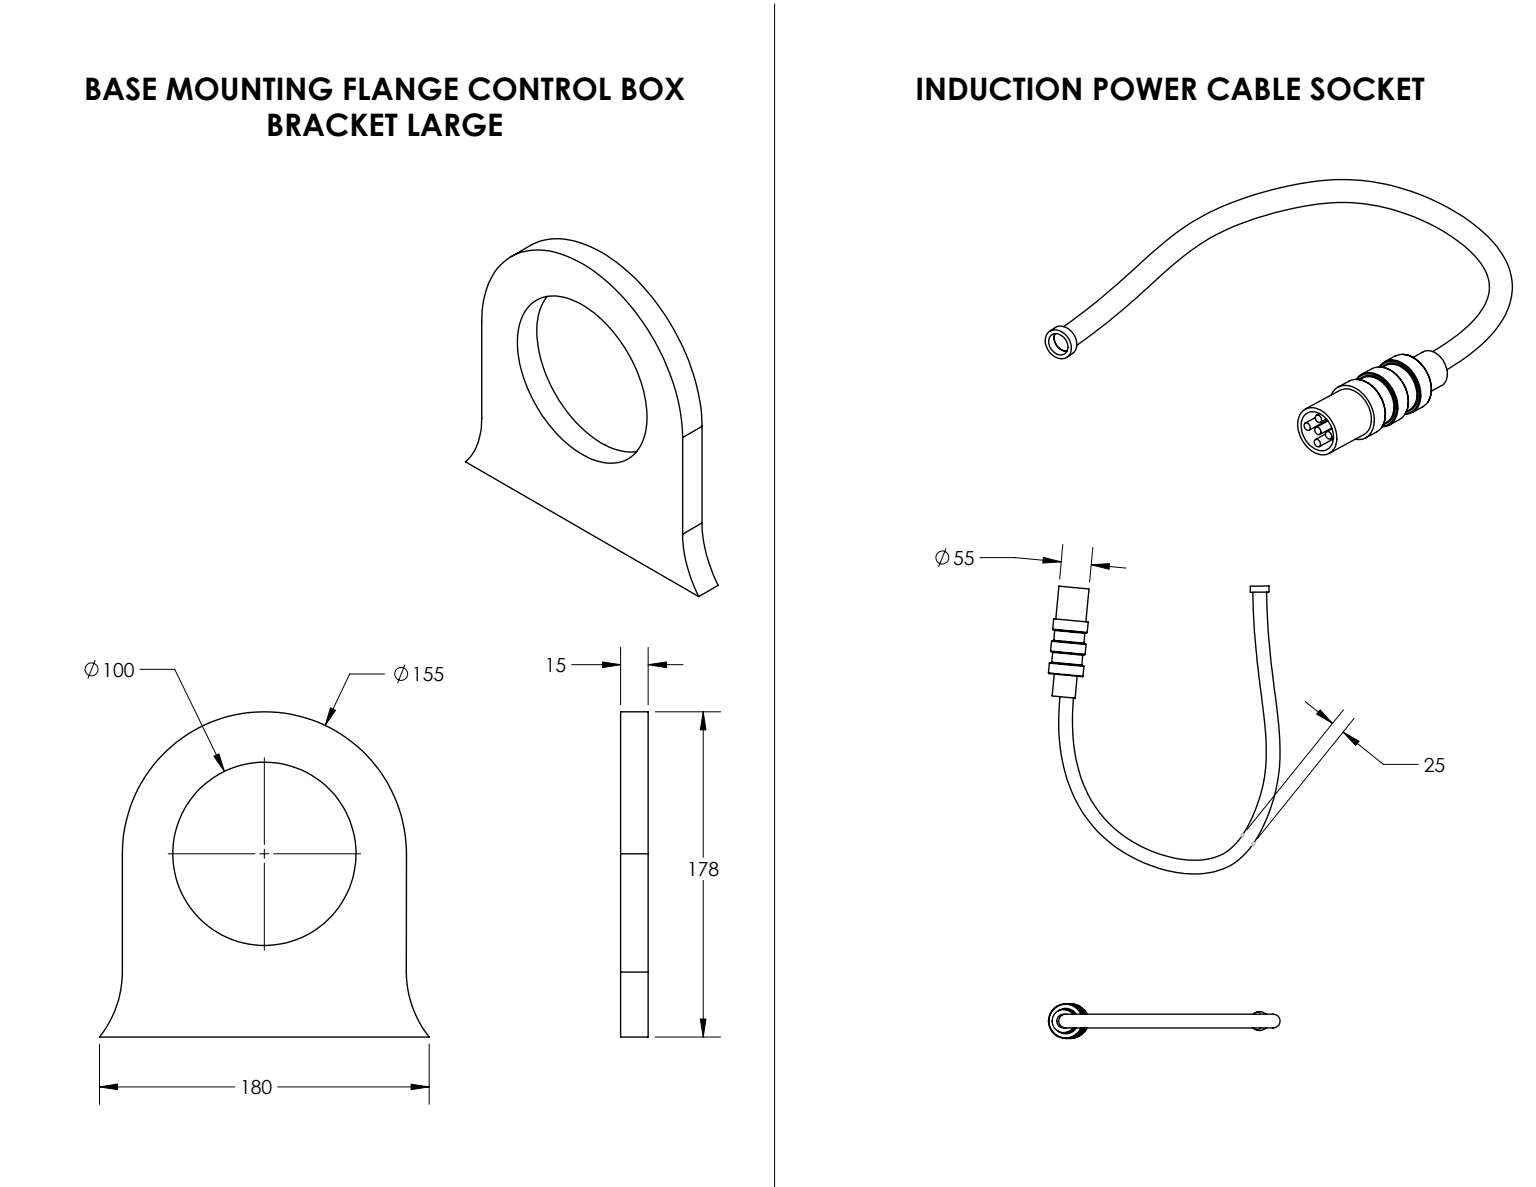
ISO-10303-21;
HEADER;
FILE_DESCRIPTION (('STEP AP214'),
    '1' );
FILE_NAME ('Base Mounting Flange Control Box Bracket large.step',
    '2026-10-28T18:30:06',
    ( '' ),
    ( '' ),
    'SwSTEP 2.0',
    'SolidWorks 2024',
    '' );
FILE_SCHEMA (( 'AUTOMOTIVE_DESIGN' ));
ENDSEC;

DATA;
#28=VECTOR ( 'NONE', #1957, 1000.000000000000114 ) ;
#31=DIRECTION ( 'NONE',  ( 0.000000000000000000, 1.000000000000000000, 0.000000000000000000 ) ) ;
#39=ORIENTED_EDGE ( 'NONE', *, *, #4059, .T. ) ;
#42=AXIS2_PLACEMENT_3D ( 'NONE', #2101, #4638, #4224 ) ;
#54=SHAPE_REPRESENTATION_RELATIONSHIP ( 'NONE' , 'NONE' ,  #825, #4179 ) ;
#57=EDGE_CURVE ( 'NONE', #2668, #1622, #1040, .T. ) ;
#90=ADVANCED_FACE ( 'NONE', ( #1835, #4370 ), #3525, .T. ) ;
#123=CARTESIAN_POINT ( 'NONE',  ( 29.23877717791899400, 15.00000000000001421, -10.40386589866737488 ) ) ;
#142=FACE_OUTER_BOUND ( 'NONE', #4109, .T. ) ;
#153=VECTOR ( 'NONE', #3723, 1000.000000000000000 ) ;
#184=DIRECTION ( 'NONE',  ( 0.000000000000000000, -1.000000000000000000, 0.000000000000000000 ) ) ;
#185=DIRECTION ( 'NONE',  ( -5.551115123125785167E-17, 0.000000000000000000, -1.000000000000000000 ) ) ;
#197=VECTOR ( 'NONE', #4836, 1000.000000000000000 ) ;
#202=DIRECTION ( 'NONE',  ( 6.938893903907233308E-17, 0.000000000000000000, 1.000000000000000000 ) ) ;
#208=CARTESIAN_POINT ( 'NONE',  ( 102.9433289385998478, 15.00000000000001421, 135.9081080810072137 ) ) ;
#225=DIRECTION ( 'NONE',  ( 6.938893903907233308E-17, 0.000000000000000000, 1.000000000000000000 ) ) ;
#226=EDGE_CURVE ( 'NONE', #1002, #2668, #2706, .T. ) ;
#228=EDGE_CURVE ( 'NONE', #5171, #2162, #3633, .T. ) ;
#243=CARTESIAN_POINT ( 'NONE',  ( -66.30461487616335603, 15.00000000000001421, 161.8139267001887447 ) ) ;
#269=DIRECTION ( 'NONE',  ( 0.000000000000000000, 0.000000000000000000, -1.000000000000000000 ) ) ;
#285=AXIS2_PLACEMENT_3D ( 'NONE', #400, #2072, #1734 ) ;
#298=EDGE_CURVE ( 'NONE', #1751, #1002, #1747, .T. ) ;
#323=ORIENTED_EDGE ( 'NONE', *, *, #228, .T. ) ;
#334=EDGE_CURVE ( 'NONE', #2890, #2427, #2526, .T. ) ;
#367=DIRECTION ( 'NONE',  ( 0.000000000000000000, 0.000000000000000000, -1.000000000000000000 ) ) ;
#368=DIRECTION ( 'NONE',  ( 0.000000000000000000, -1.000000000000000000, 0.000000000000000000 ) ) ;
#400=CARTESIAN_POINT ( 'NONE',  ( 29.23877717791899755, 15.00000000000001421, 67.09613410133263756 ) ) ;
#407=DIRECTION ( 'NONE',  ( 0.000000000000000000, 1.000000000000000000, 0.000000000000000000 ) ) ;
#419=CARTESIAN_POINT ( 'NONE',  ( 29.23877717791899755, 15.00000000000001421, 67.09613410133263756 ) ) ;
#456=CARTESIAN_POINT ( 'NONE',  ( 29.23877717791900466, 15.00000000000001421, 117.0961341013325949 ) ) ;
#458=FACE_OUTER_BOUND ( 'NONE', #2128, .T. ) ;
#460=EDGE_CURVE ( 'NONE', #2116, #2668, #3869, .T. ) ;
#474=ORIENTED_EDGE ( 'NONE', *, *, #2339, .F. ) ;
#500=ORIENTED_EDGE ( 'NONE', *, *, #5068, .F. ) ;
#519=ORIENTED_EDGE ( 'NONE', *, *, #1198, .T. ) ;
#529=CARTESIAN_POINT ( 'NONE',  ( 29.23877717791899755, 15.00000000000001421, 67.09613410133263756 ) ) ;
#530=EDGE_CURVE ( 'NONE', #606, #5098, #1451, .T. ) ;
#582=CYLINDRICAL_SURFACE ( 'NONE', #4512, 77.49999999999998579 ) ;
#590=ORIENTED_EDGE ( 'NONE', *, *, #226, .F. ) ;
#597=DIRECTION ( 'NONE',  ( 0.05689159511111528678, 0.000000000000000000, -0.9983803615885644689 ) ) ;
#602=ORIENTED_EDGE ( 'NONE', *, *, #2737, .T. ) ;
#604=DIRECTION ( 'NONE',  ( -4.476705744456277327E-17, 0.000000000000000000, -1.000000000000000000 ) ) ;
#606=VERTEX_POINT ( 'NONE', #3188 ) ;
#608=CARTESIAN_POINT ( 'NONE',  ( 29.23877717791899755, 15.00000000000001421, 67.09613410133263756 ) ) ;
#625=ORIENTED_EDGE ( 'NONE', *, *, #460, .F. ) ;
#643=ORIENTED_EDGE ( 'NONE', *, *, #2742, .F. ) ;
#663=DIRECTION ( 'NONE',  ( 0.000000000000000000, -1.000000000000000000, -0.000000000000000000 ) ) ;
#706=EDGE_LOOP ( 'NONE', ( #2402, #1700, #643, #922 ) ) ;
#708=EDGE_LOOP ( 'NONE', ( #3884, #2629, #2702, #889 ) ) ;
#715=CIRCLE ( 'NONE', #1161, 56.63911695420845405 ) ;
#746=FACE_BOUND ( 'NONE', #3021, .T. ) ;
#775=UNCERTAINTY_MEASURE_WITH_UNIT (LENGTH_MEASURE( 1.000000000000000082E-05 ), #2148, 'distance_accuracy_value', 'NONE');
#796=EDGE_CURVE ( 'NONE', #2890, #3556, #4181, .T. ) ;
#802=DIRECTION ( 'NONE',  ( -6.938893903907233308E-17, 0.000000000000000000, -1.000000000000000000 ) ) ;
#810=DIRECTION ( 'NONE',  ( 0.000000000000000000, -1.000000000000000000, 0.000000000000000000 ) ) ;
#825=SHAPE_REPRESENTATION ( 'Base Mounting Flange Control Box Bracket large', ( #2926 ), #1963 ) ;
#835=PRODUCT ( 'Base Mounting Flange Control Box Bracket large', 'Base Mounting Flange Control Box Bracket large', '', ( #4423 ) ) ;
#845=DIRECTION ( 'NONE',  ( 4.476705744456277327E-17, 0.000000000000000000, 1.000000000000000000 ) ) ;
#889=ORIENTED_EDGE ( 'NONE', *, *, #4257, .F. ) ;
#890=ORIENTED_EDGE ( 'NONE', *, *, #5426, .F. ) ;
#905=AXIS2_PLACEMENT_3D ( 'NONE', #4213, #4650, #2237 ) ;
#914=AXIS2_PLACEMENT_3D ( 'NONE', #2171, #3387, #4641 ) ;
#922=ORIENTED_EDGE ( 'NONE', *, *, #4994, .F. ) ;
#935=ADVANCED_FACE ( 'NONE', ( #3434 ), #5172, .F. ) ;
#937=CARTESIAN_POINT ( 'NONE',  ( 29.23877717791899400, 0.000000000000000000, -10.40386589866737488 ) ) ;
#948=DIRECTION ( 'NONE',  ( 0.05689159511111530065, 0.000000000000000000, -0.9983803615885645799 ) ) ;
#959=DIRECTION ( 'NONE',  ( 0.000000000000000000, 0.000000000000000000, 1.000000000000000000 ) ) ;
#1002=VERTEX_POINT ( 'NONE', #1518 ) ;
#1006=VECTOR ( 'NONE', #5359, 1000.000000000000000 ) ;
#1009=AXIS2_PLACEMENT_3D ( 'NONE', #4115, #368, #802 ) ;
#1016=DIRECTION ( 'NONE',  ( 0.000000000000000000, -1.000000000000000000, -0.000000000000000000 ) ) ;
#1040=LINE ( 'NONE', #1062, #2701 ) ;
#1044=ORIENTED_EDGE ( 'NONE', *, *, #796, .F. ) ;
#1055=AXIS2_PLACEMENT_3D ( 'NONE', #1273, #3419, #2996 ) ;
#1062=CARTESIAN_POINT ( 'NONE',  ( 102.9433289385998478, 0.000000000000000000, 135.9081080810072137 ) ) ;
#1084=DIRECTION ( 'NONE',  ( 0.000000000000000000, -1.000000000000000000, 0.000000000000000000 ) ) ;
#1103=DIRECTION ( 'NONE',  ( 0.000000000000000000, 1.000000000000000000, 0.000000000000000000 ) ) ;
#1137=CARTESIAN_POINT ( 'NONE',  ( -66.30461487616335603, 15.00000000000001421, 161.8139267001887447 ) ) ;
#1161=AXIS2_PLACEMENT_3D ( 'NONE', #3304, #2768, #1943 ) ;
#1170=CIRCLE ( 'NONE', #4070, 77.49999999999998579 ) ;
#1192=DIRECTION ( 'NONE',  ( 4.476705744456277327E-17, 0.000000000000000000, 1.000000000000000000 ) ) ;
#1198=EDGE_CURVE ( 'NONE', #1846, #1622, #3771, .T. ) ;
#1223=ORIENTED_EDGE ( 'NONE', *, *, #4128, .T. ) ;
#1227=DIRECTION ( 'NONE',  ( 0.000000000000000000, 1.000000000000000000, 0.000000000000000000 ) ) ;
#1237=ORIENTED_EDGE ( 'NONE', *, *, #3823, .T. ) ;
#1249=AXIS2_PLACEMENT_3D ( 'NONE', #4787, #1103, #225 ) ;
#1250=ADVANCED_FACE ( 'NONE', ( #4168 ), #4575, .F. ) ;
#1273=CARTESIAN_POINT ( 'NONE',  ( 29.23877717791899755, 15.00000000000001421, 67.09613410133263756 ) ) ;
#1290=VECTOR ( 'NONE', #4285, 1000.000000000000000 ) ;
#1292=ORIENTED_EDGE ( 'NONE', *, *, #5426, .T. ) ;
#1330=CARTESIAN_POINT ( 'NONE',  ( -66.30461487616335603, 15.00000000000001421, 161.8139267001887447 ) ) ;
#1336=EDGE_CURVE ( 'NONE', #2924, #3703, #1940, .T. ) ;
#1347=DIRECTION ( 'NONE',  ( 1.000000000000000000, 0.000000000000000000, 0.000000000000000000 ) ) ;
#1370=VECTOR ( 'NONE', #1084, 1000.000000000000000 ) ;
#1414=DIRECTION ( 'NONE',  ( -0.9983803615885644689, 0.000000000000000000, -0.05689159511111529371 ) ) ;
#1451=LINE ( 'NONE', #5129, #1290 ) ;
#1464=ORIENTED_EDGE ( 'NONE', *, *, #460, .T. ) ;
#1487=ORIENTED_EDGE ( 'NONE', *, *, #530, .T. ) ;
#1488=CARTESIAN_POINT ( 'NONE',  ( 29.23877717791899400, 15.00000000000001421, -10.40386589866734646 ) ) ;
#1516=ORIENTED_EDGE ( 'NONE', *, *, #2075, .F. ) ;
#1518=CARTESIAN_POINT ( 'NONE',  ( 113.4038502097781276, 0.000000000000000000, 172.0544138201894668 ) ) ;
#1535=EDGE_CURVE ( 'NONE', #4186, #606, #3442, .T. ) ;
#1559=DIRECTION ( 'NONE',  ( 0.05689159511111528678, 0.000000000000000000, -0.9983803615885644689 ) ) ;
#1615=AXIS2_PLACEMENT_3D ( 'NONE', #3562, #663, #4833 ) ;
#1622=VERTEX_POINT ( 'NONE', #3476 ) ;
#1654=VERTEX_POINT ( 'NONE', #937 ) ;
#1673=CIRCLE ( 'NONE', #3009, 49.99999999999996447 ) ;
#1685=CARTESIAN_POINT ( 'NONE',  ( -66.30461487616335603, 0.000000000000000000, 161.8139267001887447 ) ) ;
#1698=AXIS2_PLACEMENT_3D ( 'NONE', #3408, #407, #4198 ) ;
#1700=ORIENTED_EDGE ( 'NONE', *, *, #334, .T. ) ;
#1720=CARTESIAN_POINT ( 'NONE',  ( 29.23877717791899400, 15.00000000000001421, 17.09613410133265532 ) ) ;
#1722=EDGE_CURVE ( 'NONE', #3703, #1751, #715, .T. ) ;
#1734=DIRECTION ( 'NONE',  ( -6.938893903907233308E-17, 0.000000000000000000, -1.000000000000000000 ) ) ;
#1737=VECTOR ( 'NONE', #1918, 1000.000000000000114 ) ;
#1747=LINE ( 'NONE', #1685, #5341 ) ;
#1751=VERTEX_POINT ( 'NONE', #4036 ) ;
#1756=APPLICATION_CONTEXT ( 'automotive_design' ) ;
#1774=EDGE_LOOP ( 'NONE', ( #2764, #625, #4453, #2047 ) ) ;
#1783=ORIENTED_EDGE ( 'NONE', *, *, #4151, .F. ) ;
#1792=CYLINDRICAL_SURFACE ( 'NONE', #905, 77.49999999999998579 ) ;
#1818=PLANE ( 'NONE',  #2132 ) ;
#1822=ORIENTED_EDGE ( 'NONE', *, *, #1198, .F. ) ;
#1823=ORIENTED_EDGE ( 'NONE', *, *, #57, .F. ) ;
#1835=FACE_OUTER_BOUND ( 'NONE', #4872, .T. ) ;
#1843=CARTESIAN_POINT ( 'NONE',  ( -48.13570084519476211, 15.00000000000001421, 62.68703548022115513 ) ) ;
#1846=VERTEX_POINT ( 'NONE', #4637 ) ;
#1859=CARTESIAN_POINT ( 'NONE',  ( 159.4907110033991273, 15.00000000000001421, 139.1303977902171596 ) ) ;
#1861=AXIS2_PLACEMENT_3D ( 'NONE', #2922, #3772, #4216 ) ;
#1901=FACE_OUTER_BOUND ( 'NONE', #3610, .T. ) ;
#1906=EDGE_CURVE ( 'NONE', #2162, #1002, #5040, .T. ) ;
#1918=DIRECTION ( 'NONE',  ( 0.9983803615885644689, 0.000000000000000000, 0.05689159511111529371 ) ) ;
#1940=LINE ( 'NONE', #3574, #1370 ) ;
#1943=DIRECTION ( 'NONE',  ( 0.000000000000000000, 0.000000000000000000, -1.000000000000000000 ) ) ;
#1957=DIRECTION ( 'NONE',  ( -0.05689159511111523820, 0.000000000000000000, 0.9983803615885644689 ) ) ;
#1963=( GEOMETRIC_REPRESENTATION_CONTEXT ( 3 ) GLOBAL_UNCERTAINTY_ASSIGNED_CONTEXT ( ( #775 ) ) GLOBAL_UNIT_ASSIGNED_CONTEXT ( ( #2148, #4210, #4671 ) ) REPRESENTATION_CONTEXT ( 'NONE', 'WORKASPACE' ) );
#1978=CARTESIAN_POINT ( 'NONE',  ( 29.23877717791900466, 15.00000000000001421, 117.0961341013326233 ) ) ;
#2019=PRODUCT_DEFINITION_SHAPE ( 'NONE', 'NONE',  #4505 ) ;
#2029=CARTESIAN_POINT ( 'NONE',  ( 102.9433289385998478, 15.00000000000001421, 135.9081080810072137 ) ) ;
#2047=ORIENTED_EDGE ( 'NONE', *, *, #1906, .T. ) ;
#2072=DIRECTION ( 'NONE',  ( 0.000000000000000000, -1.000000000000000000, 0.000000000000000000 ) ) ;
#2075=EDGE_CURVE ( 'NONE', #3556, #2890, #1673, .T. ) ;
#2092=AXIS2_PLACEMENT_3D ( 'NONE', #4125, #5263, #2359 ) ;
#2101=CARTESIAN_POINT ( 'NONE',  ( -108.3530091724271358, 15.00000000000001421, 123.8676211295743599 ) ) ;
#2109=PLANE ( 'NONE',  #914 ) ;
#2116=VERTEX_POINT ( 'NONE', #3653 ) ;
#2128=EDGE_LOOP ( 'NONE', ( #4087, #1822, #5213, #1464 ) ) ;
#2132=AXIS2_PLACEMENT_3D ( 'NONE', #1843, #4431, #4378 ) ;
#2148=( LENGTH_UNIT ( ) NAMED_UNIT ( * ) SI_UNIT ( .MILLI., .METRE. ) );
#2162=VERTEX_POINT ( 'NONE', #2759 ) ;
#2171=CARTESIAN_POINT ( 'NONE',  ( 102.9433289385998478, 15.00000000000001421, 135.9081080810072137 ) ) ;
#2183=CARTESIAN_POINT ( 'NONE',  ( 102.9433289385998478, 0.000000000000000000, 135.9081080810072137 ) ) ;
#2237=DIRECTION ( 'NONE',  ( -4.476705744456277327E-17, 0.000000000000000000, -1.000000000000000000 ) ) ;
#2240=FACE_OUTER_BOUND ( 'NONE', #4377, .T. ) ;
#2242=ORIENTED_EDGE ( 'NONE', *, *, #1336, .T. ) ;
#2261=CLOSED_SHELL ( 'NONE', ( #2421, #4698, #4942, #90, #2946, #935, #2985, #3580, #2620, #2704, #1250 ) ) ;
#2263=ORIENTED_EDGE ( 'NONE', *, *, #530, .F. ) ;
#2280=ORIENTED_EDGE ( 'NONE', *, *, #4059, .F. ) ;
#2297=CARTESIAN_POINT ( 'NONE',  ( -51.80562710762752232, 15.00000000000001421, 127.0899108387844336 ) ) ;
#2332=SHAPE_DEFINITION_REPRESENTATION ( #2019, #825 ) ;
#2339=EDGE_CURVE ( 'NONE', #1622, #1654, #4239, .T. ) ;
#2340=CARTESIAN_POINT ( 'NONE',  ( -48.13570084519476211, 15.00000000000001421, 62.68703548022115513 ) ) ;
#2358=FACE_OUTER_BOUND ( 'NONE', #1774, .T. ) ;
#2359=DIRECTION ( 'NONE',  ( 0.000000000000000000, 0.000000000000000000, 1.000000000000000000 ) ) ;
#2380=ORIENTED_EDGE ( 'NONE', *, *, #298, .F. ) ;
#2400=AXIS2_PLACEMENT_3D ( 'NONE', #3892, #4310, #202 ) ;
#2402=ORIENTED_EDGE ( 'NONE', *, *, #2075, .T. ) ;
#2415=LINE ( 'NONE', #2029, #5211 ) ;
#2421=ADVANCED_FACE ( 'NONE', ( #4169 ), #4551, .F. ) ;
#2427=VERTEX_POINT ( 'NONE', #3753 ) ;
#2487=CARTESIAN_POINT ( 'NONE',  ( 106.6132552010327288, 15.00000000000001421, 71.50523272244407735 ) ) ;
#2526=LINE ( 'NONE', #456, #2534 ) ;
#2534=VECTOR ( 'NONE', #4205, 1000.000000000000000 ) ;
#2546=CARTESIAN_POINT ( 'NONE',  ( 113.4038502097781276, 15.00000000000001421, 172.0544138201894668 ) ) ;
#2590=CIRCLE ( 'NONE', #4177, 77.49999999999998579 ) ;
#2602=ORIENTED_EDGE ( 'NONE', *, *, #1336, .F. ) ;
#2620=ADVANCED_FACE ( 'NONE', ( #4735 ), #1792, .T. ) ;
#2629=ORIENTED_EDGE ( 'NONE', *, *, #796, .T. ) ;
#2640=ORIENTED_EDGE ( 'NONE', *, *, #5068, .T. ) ;
#2668=VERTEX_POINT ( 'NONE', #2183 ) ;
#2701=VECTOR ( 'NONE', #597, 1000.000000000000227 ) ;
#2702=ORIENTED_EDGE ( 'NONE', *, *, #4994, .T. ) ;
#2704=ADVANCED_FACE ( 'NONE', ( #142 ), #1818, .F. ) ;
#2706=CIRCLE ( 'NONE', #2092, 56.63911695420812009 ) ;
#2720=DIRECTION ( 'NONE',  ( 0.000000000000000000, -1.000000000000000000, 0.000000000000000000 ) ) ;
#2732=CARTESIAN_POINT ( 'NONE',  ( -51.80562710762752232, 0.000000000000000000, 127.0899108387844336 ) ) ;
#2737=EDGE_CURVE ( 'NONE', #2162, #2116, #3545, .T. ) ;
#2742=EDGE_CURVE ( 'NONE', #5300, #2427, #5017, .T. ) ;
#2759=CARTESIAN_POINT ( 'NONE',  ( 113.4038502097781276, 15.00000000000001421, 172.0544138201894668 ) ) ;
#2764=ORIENTED_EDGE ( 'NONE', *, *, #226, .T. ) ;
#2768=DIRECTION ( 'NONE',  ( 0.000000000000000000, -1.000000000000000000, 0.000000000000000000 ) ) ;
#2791=ORIENTED_EDGE ( 'NONE', *, *, #2339, .T. ) ;
#2792=AXIS2_PLACEMENT_3D ( 'NONE', #5181, #1016, #185 ) ;
#2851=ORIENTED_EDGE ( 'NONE', *, *, #5257, .T. ) ;
#2870=ORIENTED_EDGE ( 'NONE', *, *, #228, .F. ) ;
#2890=VERTEX_POINT ( 'NONE', #1978 ) ;
#2922=CARTESIAN_POINT ( 'NONE',  ( 29.23877717791899755, 0.000000000000000000, 67.09613410133263756 ) ) ;
#2924=VERTEX_POINT ( 'NONE', #2297 ) ;
#2926=AXIS2_PLACEMENT_3D ( 'NONE', #4646, #959, #1347 ) ;
#2930=CARTESIAN_POINT ( 'NONE',  ( 29.23877717791899755, 0.000000000000000000, 67.09613410133263756 ) ) ;
#2934=( LENGTH_UNIT ( ) NAMED_UNIT ( * ) SI_UNIT ( .MILLI., .METRE. ) );
#2946=ADVANCED_FACE ( 'NONE', ( #3400 ), #5053, .F. ) ;
#2985=ADVANCED_FACE ( 'NONE', ( #2358 ), #3250, .F. ) ;
#2996=DIRECTION ( 'NONE',  ( 4.476705744456277327E-17, 0.000000000000000000, 1.000000000000000000 ) ) ;
#2997=LINE ( 'NONE', #3828, #4342 ) ;
#3009=AXIS2_PLACEMENT_3D ( 'NONE', #608, #3072, #3460 ) ;
#3021=EDGE_LOOP ( 'NONE', ( #1516, #1044 ) ) ;
#3072=DIRECTION ( 'NONE',  ( 0.000000000000000000, 1.000000000000000000, 0.000000000000000000 ) ) ;
#3080=ORIENTED_EDGE ( 'NONE', *, *, #1906, .F. ) ;
#3090=CARTESIAN_POINT ( 'NONE',  ( 159.4907110033991273, 15.00000000000001421, 139.1303977902171596 ) ) ;
#3114=MANIFOLD_SOLID_BREP ( 'Boss-Extrude1', #2261 ) ;
#3130=LINE ( 'NONE', #4744, #3548 ) ;
#3174=PLANE ( 'NONE',  #1615 ) ;
#3179=CARTESIAN_POINT ( 'NONE',  ( -48.13570084519473369, 0.000000000000000000, 62.68703548022111249 ) ) ;
#3188=CARTESIAN_POINT ( 'NONE',  ( -48.13570084519473369, 15.00000000000001421, 62.68703548022111249 ) ) ;
#3250=CYLINDRICAL_SURFACE ( 'NONE', #4593, 56.63911695420810588 ) ;
#3270=ORIENTED_EDGE ( 'NONE', *, *, #1722, .T. ) ;
#3304=CARTESIAN_POINT ( 'NONE',  ( -108.3530091724271358, 0.000000000000000000, 123.8676211295743599 ) ) ;
#3387=DIRECTION ( 'NONE',  ( -0.9983803615885645799, 0.000000000000000000, -0.05689159511111529371 ) ) ;
#3389=ORIENTED_EDGE ( 'NONE', *, *, #4128, .F. ) ;
#3400=FACE_OUTER_BOUND ( 'NONE', #4643, .T. ) ;
#3408=CARTESIAN_POINT ( 'NONE',  ( 29.23877717791899755, 15.00000000000001421, 67.09613410133263756 ) ) ;
#3419=DIRECTION ( 'NONE',  ( 0.000000000000000000, 1.000000000000000000, 0.000000000000000000 ) ) ;
#3432=EDGE_LOOP ( 'NONE', ( #4323, #3080, #2870, #4825 ) ) ;
#3434=FACE_OUTER_BOUND ( 'NONE', #3432, .T. ) ;
#3442=CIRCLE ( 'NONE', #1055, 77.49999999999998579 ) ;
#3460=DIRECTION ( 'NONE',  ( 6.938893903907233308E-17, 0.000000000000000000, 1.000000000000000000 ) ) ;
#3476=CARTESIAN_POINT ( 'NONE',  ( 106.6132552010327288, 0.000000000000000000, 71.50523272244407735 ) ) ;
#3525=PLANE ( 'NONE',  #2792 ) ;
#3531=DIRECTION ( 'NONE',  ( 0.000000000000000000, 0.000000000000000000, 1.000000000000000000 ) ) ;
#3539=DIRECTION ( 'NONE',  ( 0.000000000000000000, -1.000000000000000000, 0.000000000000000000 ) ) ;
#3545=CIRCLE ( 'NONE', #3886, 56.63911695420812009 ) ;
#3548=VECTOR ( 'NONE', #3539, 1000.000000000000000 ) ;
#3549=STYLED_ITEM('',(#5444),#3114);
#3556=VERTEX_POINT ( 'NONE', #1720 ) ;
#3562=CARTESIAN_POINT ( 'NONE',  ( -108.3530091724271358, 15.00000000000001421, 123.8676211295743599 ) ) ;
#3574=CARTESIAN_POINT ( 'NONE',  ( -51.80562710762752232, 15.00000000000001421, 127.0899108387844336 ) ) ;
#3580=ADVANCED_FACE ( 'NONE', ( #458 ), #2109, .F. ) ;
#3610=EDGE_LOOP ( 'NONE', ( #1223, #323, #602, #1237, #1292, #3616, #4219 ) ) ;
#3614=LINE ( 'NONE', #2340, #28 ) ;
#3616=ORIENTED_EDGE ( 'NONE', *, *, #1535, .T. ) ;
#3633=LINE ( 'NONE', #243, #1737 ) ;
#3653=CARTESIAN_POINT ( 'NONE',  ( 102.9433289385998478, 15.00000000000001421, 135.9081080810072137 ) ) ;
#3703=VERTEX_POINT ( 'NONE', #2732 ) ;
#3723=DIRECTION ( 'NONE',  ( 0.000000000000000000, -1.000000000000000000, 0.000000000000000000 ) ) ;
#3742=DIRECTION ( 'NONE',  ( 0.9983803615885644689, 0.000000000000000000, 0.05689159511111529371 ) ) ;
#3753=CARTESIAN_POINT ( 'NONE',  ( 29.23877717791900466, 0.000000000000000000, 117.0961341013326233 ) ) ;
#3771=LINE ( 'NONE', #2487, #153 ) ;
#3772=DIRECTION ( 'NONE',  ( 0.000000000000000000, 1.000000000000000000, 0.000000000000000000 ) ) ;
#3779=( NAMED_UNIT ( * ) SI_UNIT ( $, .STERADIAN. ) SOLID_ANGLE_UNIT ( ) );
#3816=AXIS2_PLACEMENT_3D ( 'NONE', #1330, #948, #1414 ) ;
#3823=EDGE_CURVE ( 'NONE', #2116, #1846, #2415, .T. ) ;
#3828=CARTESIAN_POINT ( 'NONE',  ( -48.13570084519476211, 0.000000000000000000, 62.68703548022115513 ) ) ;
#3869=LINE ( 'NONE', #208, #4631 ) ;
#3881=DIRECTION ( 'NONE',  ( 0.000000000000000000, -1.000000000000000000, 0.000000000000000000 ) ) ;
#3884=ORIENTED_EDGE ( 'NONE', *, *, #334, .F. ) ;
#3886=AXIS2_PLACEMENT_3D ( 'NONE', #3090, #2720, #3531 ) ;
#3892=CARTESIAN_POINT ( 'NONE',  ( 29.23877717791899755, 0.000000000000000000, 67.09613410133263756 ) ) ;
#3900=( GEOMETRIC_REPRESENTATION_CONTEXT ( 3 ) GLOBAL_UNCERTAINTY_ASSIGNED_CONTEXT ( ( #4084 ) ) GLOBAL_UNIT_ASSIGNED_CONTEXT ( ( #2934, #4935, #3779 ) ) REPRESENTATION_CONTEXT ( 'NONE', 'WORKASPACE' ) );
#3980=AXIS2_PLACEMENT_3D ( 'NONE', #4979, #5392, #367 ) ;
#3993=ORIENTED_EDGE ( 'NONE', *, *, #4885, .F. ) ;
#4036=CARTESIAN_POINT ( 'NONE',  ( -66.30461487616335603, 0.000000000000000000, 161.8139267001887447 ) ) ;
#4044=ORIENTED_EDGE ( 'NONE', *, *, #1722, .F. ) ;
#4052=ORIENTED_EDGE ( 'NONE', *, *, #2742, .T. ) ;
#4059=EDGE_CURVE ( 'NONE', #1654, #5098, #2590, .T. ) ;
#4070=AXIS2_PLACEMENT_3D ( 'NONE', #419, #31, #1192 ) ;
#4084=UNCERTAINTY_MEASURE_WITH_UNIT (LENGTH_MEASURE( 1.000000000000000082E-05 ), #2934, 'distance_accuracy_value', 'NONE');
#4087=ORIENTED_EDGE ( 'NONE', *, *, #57, .T. ) ;
#4109=EDGE_LOOP ( 'NONE', ( #2640, #2602, #3993, #1487 ) ) ;
#4115=CARTESIAN_POINT ( 'NONE',  ( 29.23877717791899755, 15.00000000000001421, 67.09613410133263756 ) ) ;
#4125=CARTESIAN_POINT ( 'NONE',  ( 159.4907110033991273, 0.000000000000000000, 139.1303977902171596 ) ) ;
#4128=EDGE_CURVE ( 'NONE', #2924, #5171, #5304, .T. ) ;
#4151=EDGE_CURVE ( 'NONE', #5171, #1751, #3130, .T. ) ;
#4168=FACE_OUTER_BOUND ( 'NONE', #708, .T. ) ;
#4169=FACE_OUTER_BOUND ( 'NONE', #706, .T. ) ;
#4177=AXIS2_PLACEMENT_3D ( 'NONE', #2930, #1227, #845 ) ;
#4179=ADVANCED_BREP_SHAPE_REPRESENTATION ( '', ( #3114, #2926 ), #1963 ) ;
#4181=CIRCLE ( 'NONE', #1698, 49.99999999999996447 ) ;
#4186=VERTEX_POINT ( 'NONE', #123 ) ;
#4198=DIRECTION ( 'NONE',  ( 6.938893903907233308E-17, 0.000000000000000000, 1.000000000000000000 ) ) ;
#4205=DIRECTION ( 'NONE',  ( 0.000000000000000000, -1.000000000000000000, 0.000000000000000000 ) ) ;
#4210=( NAMED_UNIT ( * ) PLANE_ANGLE_UNIT ( ) SI_UNIT ( $, .RADIAN. ) );
#4213=CARTESIAN_POINT ( 'NONE',  ( 29.23877717791899755, 15.00000000000001421, 67.09613410133263756 ) ) ;
#4214=CARTESIAN_POINT ( 'NONE',  ( 29.23877717791899400, 0.000000000000000000, 17.09613410133265532 ) ) ;
#4216=DIRECTION ( 'NONE',  ( 4.476705744456277327E-17, 0.000000000000000000, 1.000000000000000000 ) ) ;
#4219=ORIENTED_EDGE ( 'NONE', *, *, #4885, .T. ) ;
#4224=DIRECTION ( 'NONE',  ( 0.000000000000000000, 0.000000000000000000, -1.000000000000000000 ) ) ;
#4239=CIRCLE ( 'NONE', #1861, 77.49999999999998579 ) ;
#4257=EDGE_CURVE ( 'NONE', #2427, #5300, #5216, .T. ) ;
#4285=DIRECTION ( 'NONE',  ( 0.000000000000000000, -1.000000000000000000, 0.000000000000000000 ) ) ;
#4310=DIRECTION ( 'NONE',  ( 0.000000000000000000, 1.000000000000000000, 0.000000000000000000 ) ) ;
#4323=ORIENTED_EDGE ( 'NONE', *, *, #298, .T. ) ;
#4342=VECTOR ( 'NONE', #5074, 1000.000000000000114 ) ;
#4354=PRODUCT_DEFINITION_FORMATION_WITH_SPECIFIED_SOURCE ( 'ANY', '', #835, .NOT_KNOWN. ) ;
#4370=FACE_BOUND ( 'NONE', #4484, .T. ) ;
#4377=EDGE_LOOP ( 'NONE', ( #4973, #2851, #39, #2263 ) ) ;
#4378=DIRECTION ( 'NONE',  ( 0.05689159511111523820, 0.000000000000000000, -0.9983803615885644689 ) ) ;
#4420=MECHANICAL_DESIGN_GEOMETRIC_PRESENTATION_REPRESENTATION('',(#3549),#3900);
#4423=PRODUCT_CONTEXT ( 'NONE', #1756, 'mechanical' ) ;
#4431=DIRECTION ( 'NONE',  ( 0.9983803615885645799, 0.000000000000000000, 0.05689159511111524514 ) ) ;
#4453=ORIENTED_EDGE ( 'NONE', *, *, #2737, .F. ) ;
#4484=EDGE_LOOP ( 'NONE', ( #4052, #4508 ) ) ;
#4505=PRODUCT_DEFINITION ( 'UNKNOWN', '', #4354, #5337 ) ;
#4508=ORIENTED_EDGE ( 'NONE', *, *, #4257, .T. ) ;
#4512=AXIS2_PLACEMENT_3D ( 'NONE', #529, #3881, #604 ) ;
#4551=CYLINDRICAL_SURFACE ( 'NONE', #285, 49.99999999999996447 ) ;
#4575=CYLINDRICAL_SURFACE ( 'NONE', #1009, 49.99999999999996447 ) ;
#4593=AXIS2_PLACEMENT_3D ( 'NONE', #1859, #184, #269 ) ;
#4620=CARTESIAN_POINT ( 'NONE',  ( 29.23877717791899400, 15.00000000000001421, 17.09613410133267664 ) ) ;
#4631=VECTOR ( 'NONE', #4772, 1000.000000000000000 ) ;
#4637=CARTESIAN_POINT ( 'NONE',  ( 106.6132552010327288, 15.00000000000001421, 71.50523272244407735 ) ) ;
#4638=DIRECTION ( 'NONE',  ( 0.000000000000000000, -1.000000000000000000, 0.000000000000000000 ) ) ;
#4641=DIRECTION ( 'NONE',  ( -0.05689159511111528678, 0.000000000000000000, 0.9983803615885644689 ) ) ;
#4643=EDGE_LOOP ( 'NONE', ( #3270, #1783, #3389, #2242 ) ) ;
#4646=CARTESIAN_POINT ( 'NONE',  ( 0.000000000000000000, 0.000000000000000000, 0.000000000000000000 ) ) ;
#4650=DIRECTION ( 'NONE',  ( 0.000000000000000000, -1.000000000000000000, 0.000000000000000000 ) ) ;
#4668=VECTOR ( 'NONE', #810, 1000.000000000000000 ) ;
#4671=( NAMED_UNIT ( * ) SI_UNIT ( $, .STERADIAN. ) SOLID_ANGLE_UNIT ( ) );
#4698=ADVANCED_FACE ( 'NONE', ( #2240 ), #582, .T. ) ;
#4735=FACE_OUTER_BOUND ( 'NONE', #5083, .T. ) ;
#4744=CARTESIAN_POINT ( 'NONE',  ( -66.30461487616335603, 15.00000000000001421, 161.8139267001887447 ) ) ;
#4772=DIRECTION ( 'NONE',  ( 0.000000000000000000, -1.000000000000000000, 0.000000000000000000 ) ) ;
#4787=CARTESIAN_POINT ( 'NONE',  ( 29.23877717791899755, 0.000000000000000000, 67.09613410133263756 ) ) ;
#4805=ORIENTED_EDGE ( 'NONE', *, *, #5257, .F. ) ;
#4825=ORIENTED_EDGE ( 'NONE', *, *, #4151, .T. ) ;
#4833=DIRECTION ( 'NONE',  ( -5.551115123125785167E-17, 0.000000000000000000, -1.000000000000000000 ) ) ;
#4836=DIRECTION ( 'NONE',  ( 0.000000000000000000, -1.000000000000000000, 0.000000000000000000 ) ) ;
#4872=EDGE_LOOP ( 'NONE', ( #4044, #500, #2280, #474, #1823, #590, #2380 ) ) ;
#4885=EDGE_CURVE ( 'NONE', #606, #2924, #3614, .T. ) ;
#4935=( NAMED_UNIT ( * ) PLANE_ANGLE_UNIT ( ) SI_UNIT ( $, .RADIAN. ) );
#4942=ADVANCED_FACE ( 'NONE', ( #1901, #746 ), #3174, .F. ) ;
#4973=ORIENTED_EDGE ( 'NONE', *, *, #1535, .F. ) ;
#4979=CARTESIAN_POINT ( 'NONE',  ( -108.3530091724271358, 15.00000000000001421, 123.8676211295743599 ) ) ;
#4994=EDGE_CURVE ( 'NONE', #3556, #5300, #5049, .T. ) ;
#5017=CIRCLE ( 'NONE', #1249, 49.99999999999996447 ) ;
#5040=LINE ( 'NONE', #2546, #4668 ) ;
#5049=LINE ( 'NONE', #4620, #1006 ) ;
#5053=CYLINDRICAL_SURFACE ( 'NONE', #3980, 56.63911695420845405 ) ;
#5068=EDGE_CURVE ( 'NONE', #5098, #3703, #2997, .T. ) ;
#5074=DIRECTION ( 'NONE',  ( -0.05689159511111523820, 0.000000000000000000, 0.9983803615885644689 ) ) ;
#5083=EDGE_LOOP ( 'NONE', ( #4805, #890, #519, #2791 ) ) ;
#5098=VERTEX_POINT ( 'NONE', #3179 ) ;
#5129=CARTESIAN_POINT ( 'NONE',  ( -48.13570084519473369, 15.00000000000001421, 62.68703548022111249 ) ) ;
#5171=VERTEX_POINT ( 'NONE', #1137 ) ;
#5172=PLANE ( 'NONE',  #3816 ) ;
#5181=CARTESIAN_POINT ( 'NONE',  ( -108.3530091724271358, 0.000000000000000000, 123.8676211295743599 ) ) ;
#5211=VECTOR ( 'NONE', #1559, 1000.000000000000227 ) ;
#5213=ORIENTED_EDGE ( 'NONE', *, *, #3823, .F. ) ;
#5216=CIRCLE ( 'NONE', #2400, 49.99999999999996447 ) ;
#5249=LINE ( 'NONE', #1488, #197 ) ;
#5257=EDGE_CURVE ( 'NONE', #4186, #1654, #5249, .T. ) ;
#5263=DIRECTION ( 'NONE',  ( 0.000000000000000000, -1.000000000000000000, 0.000000000000000000 ) ) ;
#5300=VERTEX_POINT ( 'NONE', #4214 ) ;
#5304=CIRCLE ( 'NONE', #42, 56.63911695420845405 ) ;
#5337=PRODUCT_DEFINITION_CONTEXT ( 'detailed design', #5411, 'design' ) ;
#5341=VECTOR ( 'NONE', #3742, 1000.000000000000114 ) ;
#5359=DIRECTION ( 'NONE',  ( 0.000000000000000000, -1.000000000000000000, 0.000000000000000000 ) ) ;
#5392=DIRECTION ( 'NONE',  ( 0.000000000000000000, -1.000000000000000000, 0.000000000000000000 ) ) ;
#5411=APPLICATION_CONTEXT ( 'automotive_design' ) ;
#5426=EDGE_CURVE ( 'NONE', #1846, #4186, #1170, .T. ) ;
#5438=COLOUR_RGB('Dark Blue',0.08,0.2,0.34);
#5439=FILL_AREA_STYLE_COLOUR('',#5438);
#5440=FILL_AREA_STYLE('',(#5439));
#5441=SURFACE_STYLE_FILL_AREA(#5440);
#5442=SURFACE_SIDE_STYLE('',(#5441));
#5443=SURFACE_STYLE_USAGE(.BOTH.,#5442);
#5444=PRESENTATION_STYLE_ASSIGNMENT((#5443));
ENDSEC;
END-ISO-10303-21;
